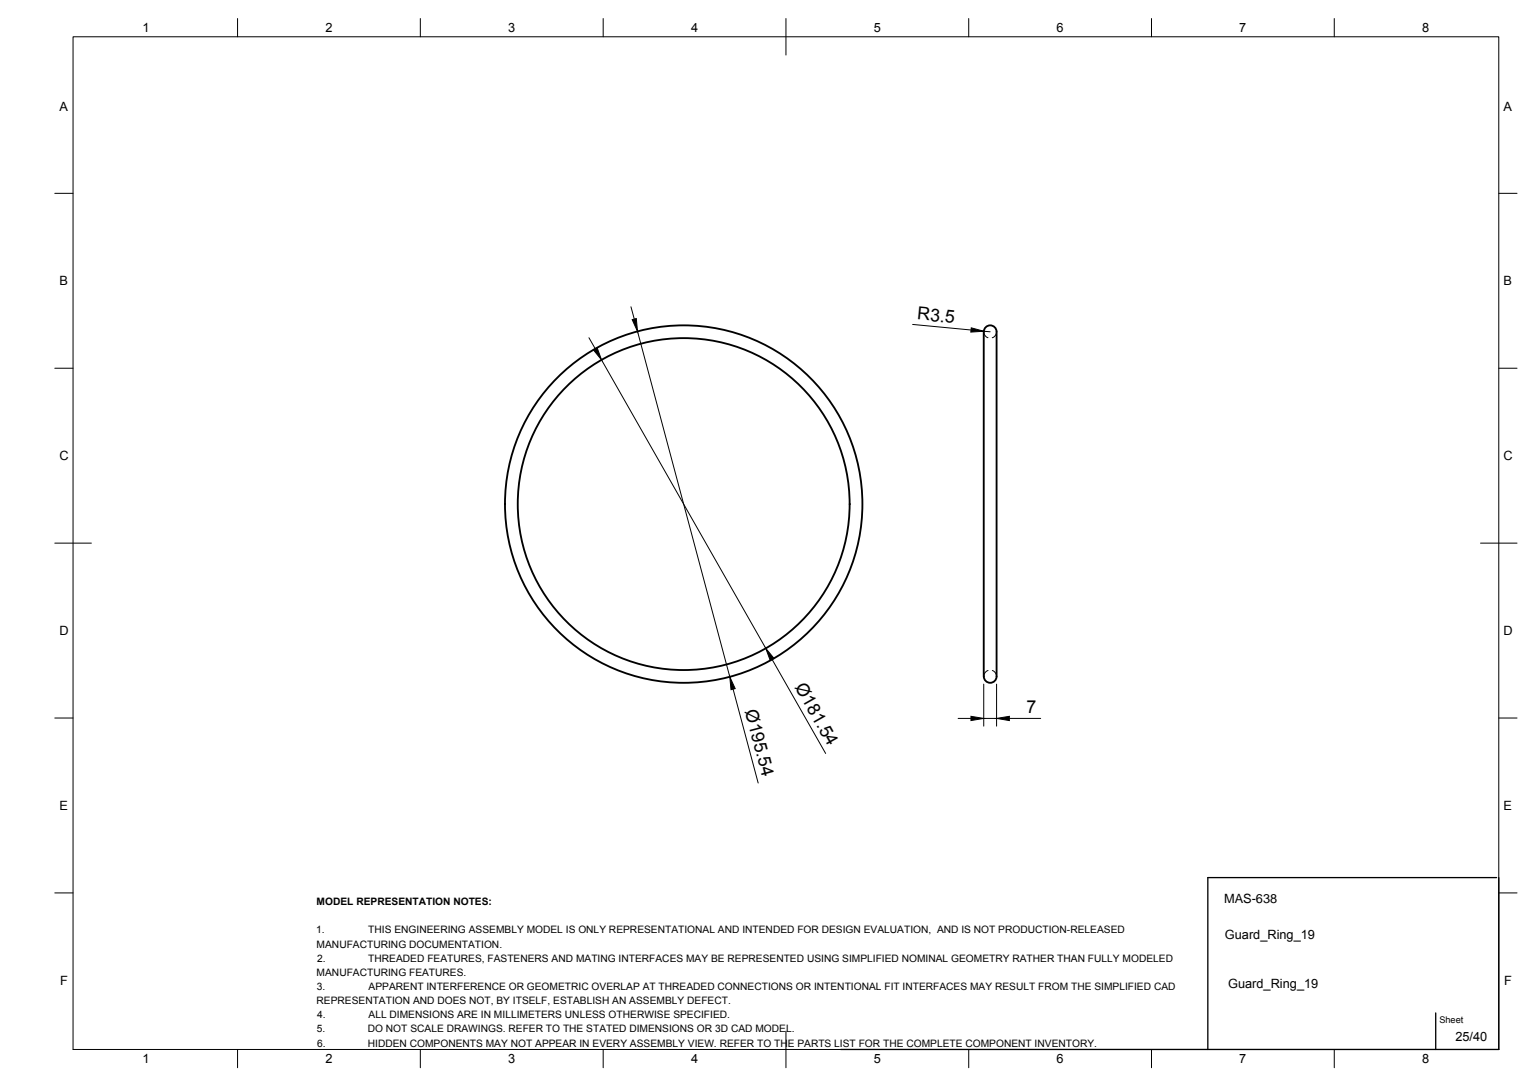
ISO-10303-21;
HEADER;
FILE_DESCRIPTION((''),'2;1');
FILE_NAME('Guard_Ring_19.step','2026-10-09T12:00:21-07:00',(''),(''),'','','');
FILE_SCHEMA (('AUTOMOTIVE_DESIGN { 1 0 10303 214 3 1 1 }'));
ENDSEC;
DATA;
#10=MECHANICAL_DESIGN_GEOMETRIC_PRESENTATION_REPRESENTATION('',(#424),#10334);
#352=SHAPE_REPRESENTATION_RELATIONSHIP('SRR','None',#10468,#384) ;
#384=ADVANCED_BREP_SHAPE_REPRESENTATION('',(#456),#10320) ;
#424=STYLED_ITEM('',(#10631),#456) ;
#456=MANIFOLD_SOLID_BREP('Body1',#3578) ;
#877=FACE_OUTER_BOUND('',#1077,.T.) ;
#1077=EDGE_LOOP('',(#2421,#2422,#2423,#2424)) ;
#1312=CIRCLE('',#4047,0.349999999999999) ;
#1313=CIRCLE('',#4048,9.07681446136679) ;
#1531=VERTEX_POINT('',#5743) ;
#1867=EDGE_CURVE('',#1531,#1531,#1312,.T.) ;
#1868=EDGE_CURVE('',#1531,#1531,#1313,.T.) ;
#2421=ORIENTED_EDGE('',*,*,#1867,.F.) ;
#2422=ORIENTED_EDGE('',*,*,#1868,.T.) ;
#2423=ORIENTED_EDGE('',*,*,#1867,.T.) ;
#2424=ORIENTED_EDGE('',*,*,#1868,.F.) ;
#3323=TOROIDAL_SURFACE('',#4046,9.42681446136679,0.349999999999999) ;
#3385=ADVANCED_FACE('',(#877),#3323,.T.) ;
#3578=CLOSED_SHELL('',(#3385)) ;
#4045=AXIS2_PLACEMENT_3D('',#5741,#4651,#4652) ;
#4046=AXIS2_PLACEMENT_3D('',#5742,#4653,#4654) ;
#4047=AXIS2_PLACEMENT_3D('',#5744,#4655,#4656) ;
#4048=AXIS2_PLACEMENT_3D('',#5745,#4657,#4658) ;
#4651=DIRECTION('axis',(0.,0.,1.)) ;
#4652=DIRECTION('refdir',(1.,0.,0.)) ;
#4653=DIRECTION('center_axis',(-6.42891162084177E-17,-1.,-1.01883556321148E-16)) ;
#4654=DIRECTION('ref_axis',(1.,0.,0.)) ;
#4655=DIRECTION('center_axis',(0.,1.01883556321148E-16,-1.)) ;
#4656=DIRECTION('ref_axis',(-1.,0.,0.)) ;
#4657=DIRECTION('center_axis',(6.42891162084177E-17,1.,1.01883556321148E-16)) ;
#4658=DIRECTION('ref_axis',(1.,-6.42891162084177E-17,-6.55000379205715E-33)) ;
#5741=CARTESIAN_POINT('',(0.,0.,0.)) ;
#5742=CARTESIAN_POINT('Origin',(23.47768801576,64.5831179463143,68.2224337400009)) ;
#5743=CARTESIAN_POINT('',(14.4008735543932,64.5831179463143,68.2224337400009)) ;
#5744=CARTESIAN_POINT('Origin',(14.0508735543932,64.5831179463143,68.2224337400009)) ;
#5745=CARTESIAN_POINT('Origin',(23.47768801576,64.5831179463143,68.2224337400009)) ;
#10283=UNCERTAINTY_MEASURE_WITH_UNIT(LENGTH_MEASURE(0.001),#10335,
'DISTANCE_ACCURACY_VALUE',
'Maximum model space distance between geometric entities at asserted c
onnectivities') ;
#10297=UNCERTAINTY_MEASURE_WITH_UNIT(LENGTH_MEASURE(0.001),#10335,
'DISTANCE_ACCURACY_VALUE',
'Maximum model space distance between geometric entities at asserted c
onnectivities') ;
#10320=(
GEOMETRIC_REPRESENTATION_CONTEXT(3)
GLOBAL_UNCERTAINTY_ASSIGNED_CONTEXT((#10283))
GLOBAL_UNIT_ASSIGNED_CONTEXT((#10335,#10337,#10338))
REPRESENTATION_CONTEXT('','3D')
) ;
#10334=(
GEOMETRIC_REPRESENTATION_CONTEXT(3)
GLOBAL_UNCERTAINTY_ASSIGNED_CONTEXT((#10297))
GLOBAL_UNIT_ASSIGNED_CONTEXT((#10335,#10337,#10338))
REPRESENTATION_CONTEXT('','3D')
) ;
#10335=(
LENGTH_UNIT()
NAMED_UNIT(*)
SI_UNIT(.CENTI.,.METRE.)
) ;
#10337=(
NAMED_UNIT(*)
PLANE_ANGLE_UNIT()
SI_UNIT($,.RADIAN.)
) ;
#10338=(
NAMED_UNIT(*)
SI_UNIT($,.STERADIAN.)
SOLID_ANGLE_UNIT()
) ;
#10361=SHAPE_DEFINITION_REPRESENTATION(#10397,#10468) ;
#10397=PRODUCT_DEFINITION_SHAPE('',$,#10505) ;
#10468=SHAPE_REPRESENTATION('',(#4045),#10320) ;
#10482=PRODUCT_DEFINITION_CONTEXT('part definition',#10592,'design') ;
#10505=PRODUCT_DEFINITION('Guard_Ring_19','Guard_Ring_19',#10541,#10482) ;
#10541=PRODUCT_DEFINITION_FORMATION('',$,#10616) ;
#10592=APPLICATION_CONTEXT(
'Core Data for Automotive Mechanical Design Process') ;
#10593=PRODUCT_CONTEXT('part definition',#10592,'mechanical') ;
#10616=PRODUCT('Guard_Ring_19','Guard_Ring_19',$,(#10593)) ;
#10631=PRESENTATION_STYLE_ASSIGNMENT((#10635)) ;
#10635=SURFACE_STYLE_USAGE(.BOTH.,#10639) ;
#10639=SURFACE_SIDE_STYLE('',(#10643)) ;
#10643=SURFACE_STYLE_FILL_AREA(#10647) ;
#10647=FILL_AREA_STYLE('Opaque(25,25,25)',(#10651)) ;
#10651=FILL_AREA_STYLE_COLOUR('Opaque(25,25,25)',#10655) ;
#10655=COLOUR_RGB('Opaque(25,25,25)', 0.09019608, 0.27058824, 0.51372549) ;
ENDSEC;
END-ISO-10303-21;
